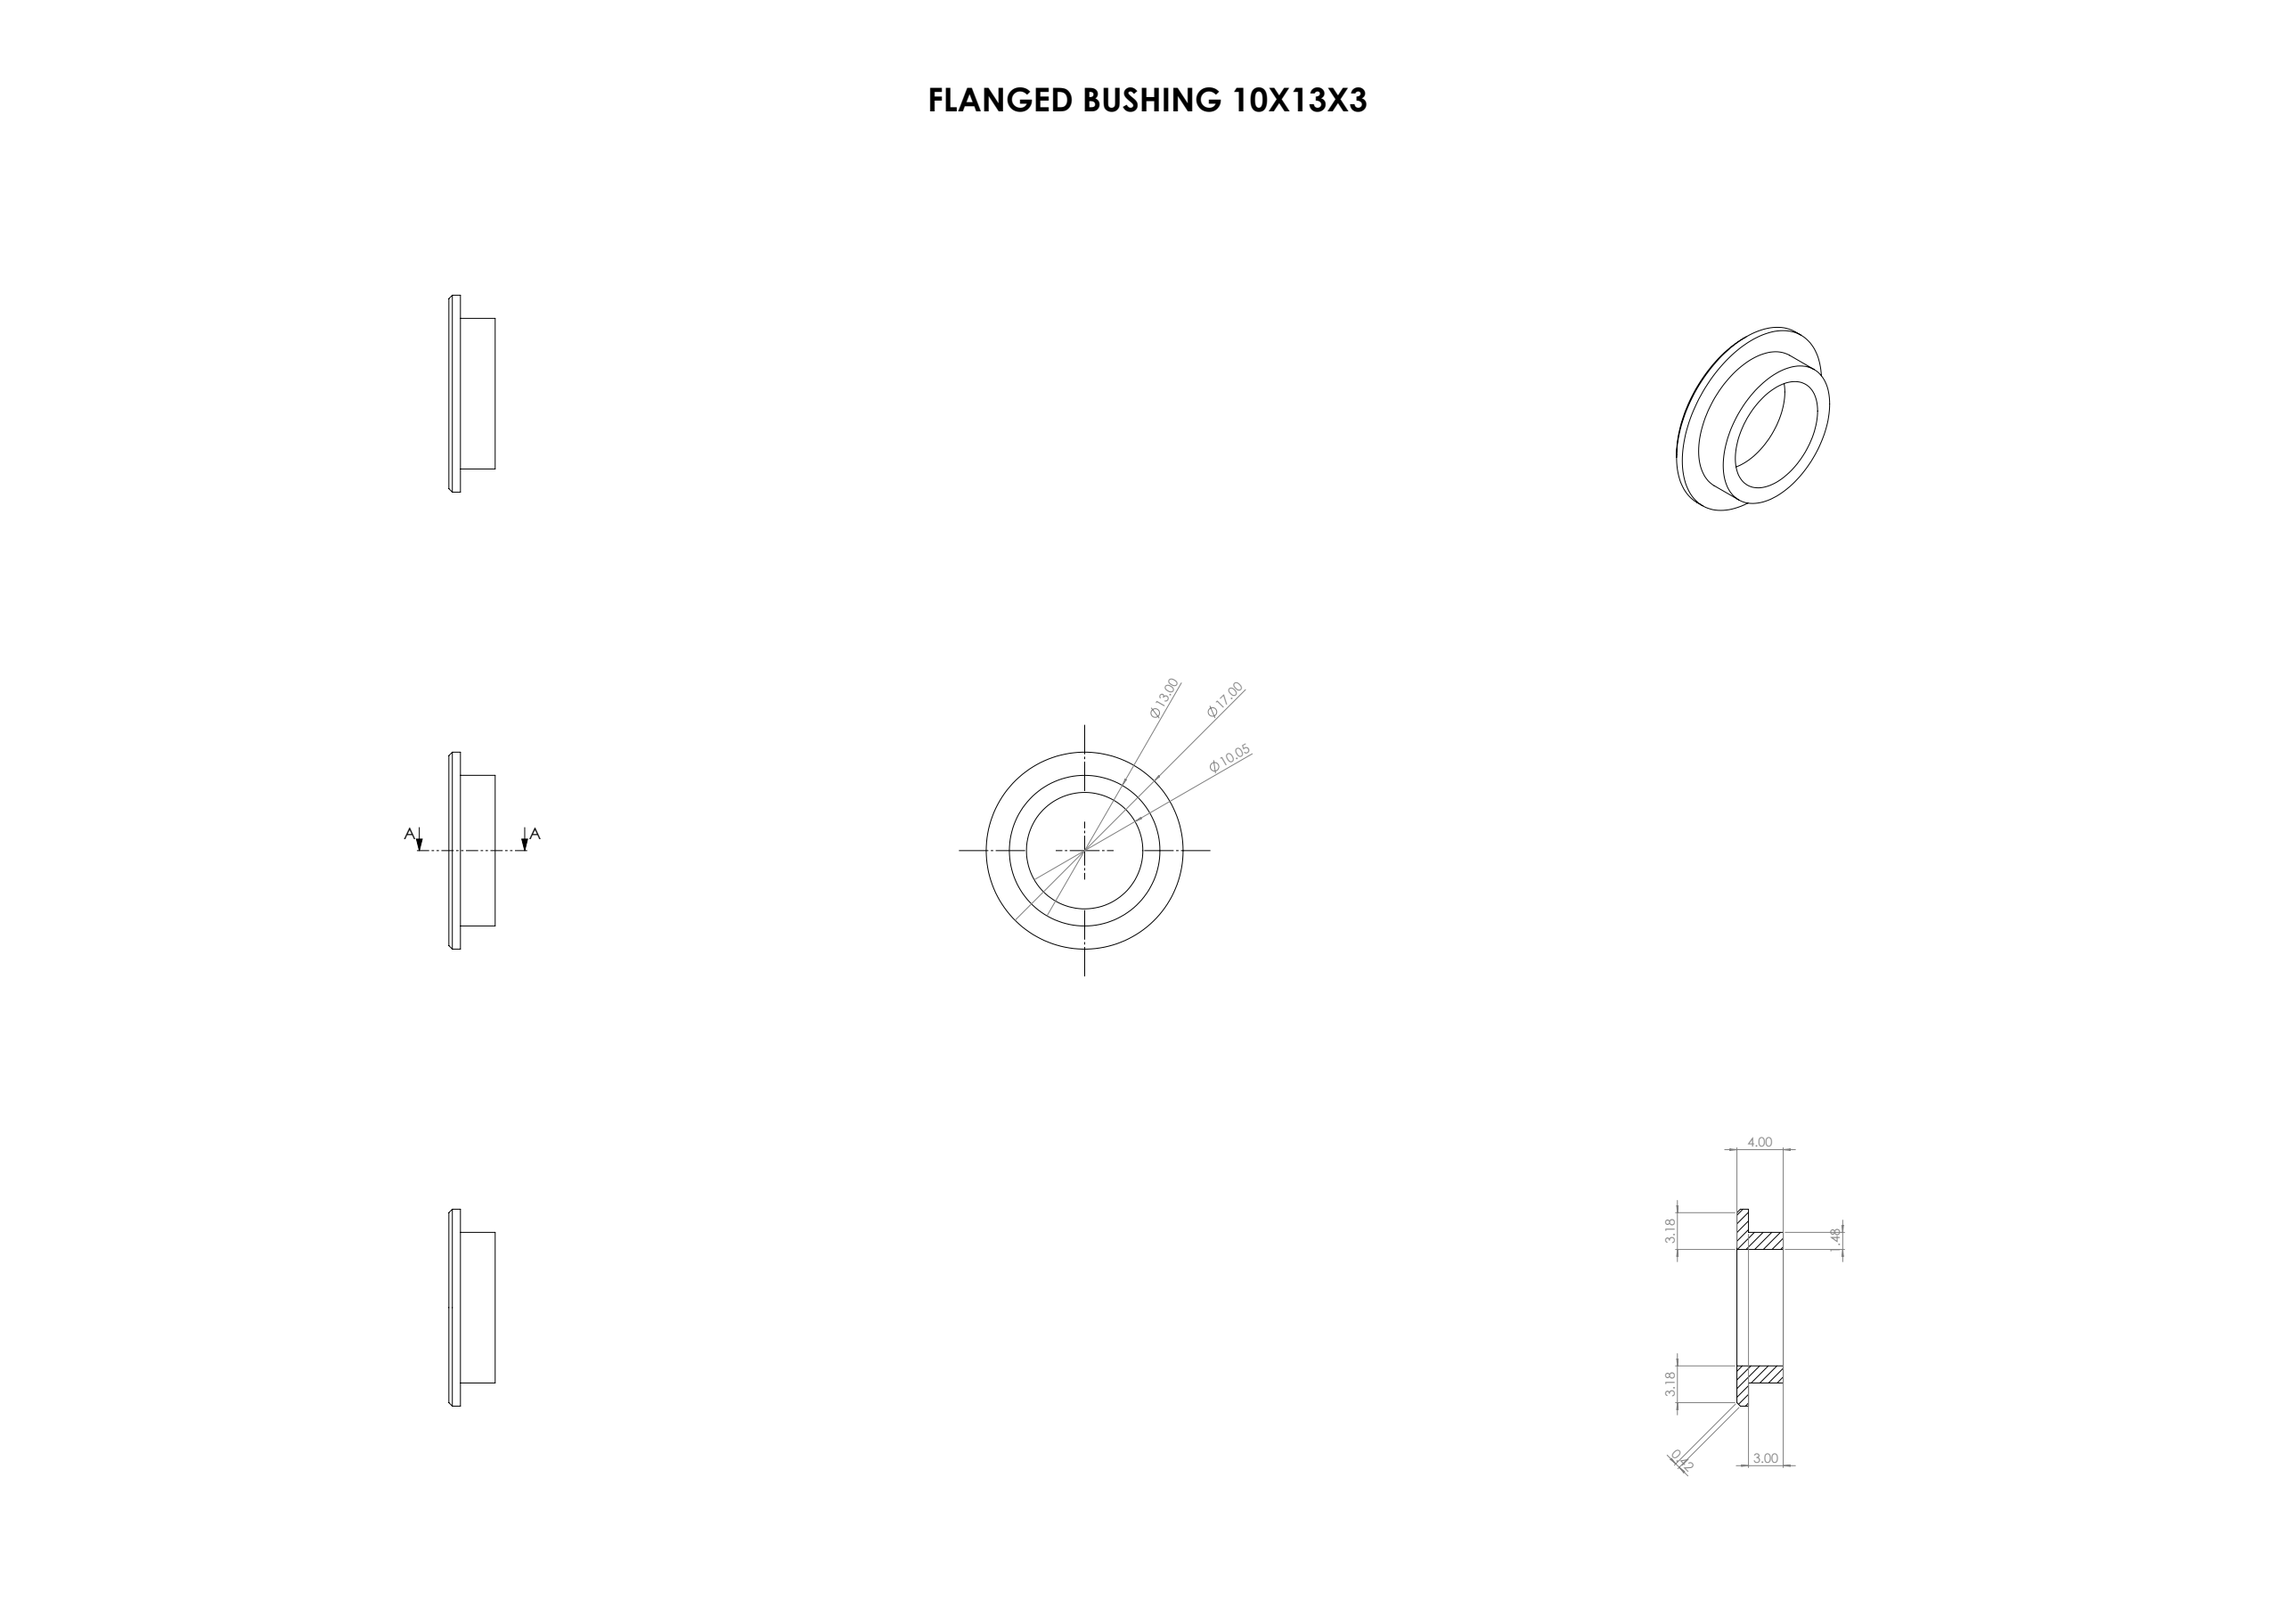
ISO-10303-21;
HEADER;
/* Generated by software containing ST-Developer
 * from STEP Tools, Inc. (www.steptools.com) 
 */

FILE_DESCRIPTION(
/* description */ (''),
/* implementation_level */ '2;1');

FILE_NAME(
/* name */ '08_Flanged_Bushing_10x13x3.step',
/* time_stamp */ '2026-10-21T01:59:45-07:00',
/* author */ (''),
/* organization */ (''),
/* preprocessor_version */ 'ST-DEVELOPER v20.2',
/* originating_system */ 'Autodesk Translation Framework v15.15.0.0',
/* authorisation */ '');

FILE_SCHEMA (('AUTOMOTIVE_DESIGN { 1 0 10303 214 3 1 1 }'));
ENDSEC;

DATA;
#10=MECHANICAL_DESIGN_GEOMETRIC_PRESENTATION_REPRESENTATION('',(#476),#18281);
#420=CONICAL_SURFACE('',#9714,8.35,0.785398163397449);
#445=SHAPE_REPRESENTATION_RELATIONSHIP('SRR','None',#18347,#458);
#458=ADVANCED_BREP_SHAPE_REPRESENTATION('',(#489),#18276);
#476=STYLED_ITEM('',(#18488),#489);
#489=MANIFOLD_SOLID_BREP('Body1',#9093);
#530=CYLINDRICAL_SURFACE('',#9720,8.5);
#531=CYLINDRICAL_SURFACE('',#9722,5.025);
#532=CYLINDRICAL_SURFACE('',#9726,6.5);
#620=FACE_BOUND('',#1771,.T.);
#621=FACE_BOUND('',#1775,.T.);
#622=FACE_BOUND('',#1778,.T.);
#755=CIRCLE('',#9715,8.5);
#756=CIRCLE('',#9716,8.5);
#757=CIRCLE('',#9717,8.2);
#758=CIRCLE('',#9719,5.025);
#759=CIRCLE('',#9721,8.5);
#760=CIRCLE('',#9723,5.025);
#761=CIRCLE('',#9725,6.5);
#762=CIRCLE('',#9727,6.5);
#1206=FACE_OUTER_BOUND('',#1769,.T.);
#1207=FACE_OUTER_BOUND('',#1770,.T.);
#1208=FACE_OUTER_BOUND('',#1772,.T.);
#1209=FACE_OUTER_BOUND('',#1773,.T.);
#1210=FACE_OUTER_BOUND('',#1774,.T.);
#1211=FACE_OUTER_BOUND('',#1776,.T.);
#1212=FACE_OUTER_BOUND('',#1777,.T.);
#1769=EDGE_LOOP('',(#7440,#7441,#7442,#7443,#7444));
#1770=EDGE_LOOP('',(#7445));
#1771=EDGE_LOOP('',(#7446));
#1772=EDGE_LOOP('',(#7447,#7448,#7449,#7450,#7451));
#1773=EDGE_LOOP('',(#7452,#7453,#7454,#7455));
#1774=EDGE_LOOP('',(#7456));
#1775=EDGE_LOOP('',(#7457));
#1776=EDGE_LOOP('',(#7458,#7459,#7460,#7461));
#1777=EDGE_LOOP('',(#7462));
#1778=EDGE_LOOP('',(#7463));
#2567=LINE('',#14541,#3412);
#2568=LINE('',#14549,#3413);
#2569=LINE('',#14553,#3414);
#2570=LINE('',#14560,#3415);
#3412=VECTOR('',#11551,8.35);
#3413=VECTOR('',#11562,8.5);
#3414=VECTOR('',#11567,5.025);
#3415=VECTOR('',#11576,6.5);
#4161=VERTEX_POINT('',#14536);
#4162=VERTEX_POINT('',#14537);
#4163=VERTEX_POINT('',#14540);
#4164=VERTEX_POINT('',#14544);
#4165=VERTEX_POINT('',#14547);
#4166=VERTEX_POINT('',#14551);
#4167=VERTEX_POINT('',#14555);
#4168=VERTEX_POINT('',#14558);
#5292=EDGE_CURVE('',#4161,#4162,#755,.T.);
#5293=EDGE_CURVE('',#4162,#4161,#756,.T.);
#5294=EDGE_CURVE('',#4161,#4163,#2567,.T.);
#5295=EDGE_CURVE('',#4163,#4163,#757,.T.);
#5296=EDGE_CURVE('',#4164,#4164,#758,.T.);
#5297=EDGE_CURVE('',#4165,#4165,#759,.T.);
#5298=EDGE_CURVE('',#4165,#4162,#2568,.T.);
#5299=EDGE_CURVE('',#4166,#4166,#760,.T.);
#5300=EDGE_CURVE('',#4166,#4164,#2569,.T.);
#5301=EDGE_CURVE('',#4167,#4167,#761,.T.);
#5302=EDGE_CURVE('',#4168,#4168,#762,.T.);
#5303=EDGE_CURVE('',#4168,#4167,#2570,.T.);
#7440=ORIENTED_EDGE('',*,*,#5292,.T.);
#7441=ORIENTED_EDGE('',*,*,#5293,.T.);
#7442=ORIENTED_EDGE('',*,*,#5294,.T.);
#7443=ORIENTED_EDGE('',*,*,#5295,.T.);
#7444=ORIENTED_EDGE('',*,*,#5294,.F.);
#7445=ORIENTED_EDGE('',*,*,#5295,.F.);
#7446=ORIENTED_EDGE('',*,*,#5296,.T.);
#7447=ORIENTED_EDGE('',*,*,#5297,.F.);
#7448=ORIENTED_EDGE('',*,*,#5298,.T.);
#7449=ORIENTED_EDGE('',*,*,#5292,.F.);
#7450=ORIENTED_EDGE('',*,*,#5293,.F.);
#7451=ORIENTED_EDGE('',*,*,#5298,.F.);
#7452=ORIENTED_EDGE('',*,*,#5299,.T.);
#7453=ORIENTED_EDGE('',*,*,#5300,.T.);
#7454=ORIENTED_EDGE('',*,*,#5296,.F.);
#7455=ORIENTED_EDGE('',*,*,#5300,.F.);
#7456=ORIENTED_EDGE('',*,*,#5297,.T.);
#7457=ORIENTED_EDGE('',*,*,#5301,.F.);
#7458=ORIENTED_EDGE('',*,*,#5302,.F.);
#7459=ORIENTED_EDGE('',*,*,#5303,.T.);
#7460=ORIENTED_EDGE('',*,*,#5301,.T.);
#7461=ORIENTED_EDGE('',*,*,#5303,.F.);
#7462=ORIENTED_EDGE('',*,*,#5302,.T.);
#7463=ORIENTED_EDGE('',*,*,#5299,.F.);
#8476=PLANE('',#9718);
#8477=PLANE('',#9724);
#8478=PLANE('',#9728);
#8927=ADVANCED_FACE('',(#1206),#420,.T.);
#8928=ADVANCED_FACE('',(#1207,#620),#8476,.T.);
#8929=ADVANCED_FACE('',(#1208),#530,.T.);
#8930=ADVANCED_FACE('',(#1209),#531,.F.);
#8931=ADVANCED_FACE('',(#1210,#621),#8477,.T.);
#8932=ADVANCED_FACE('',(#1211),#532,.T.);
#8933=ADVANCED_FACE('',(#1212,#622),#8478,.T.);
#9093=CLOSED_SHELL('',(#8927,#8928,#8929,#8930,#8931,#8932,#8933));
#9713=AXIS2_PLACEMENT_3D('',#14534,#11543,#11544);
#9714=AXIS2_PLACEMENT_3D('',#14535,#11545,#11546);
#9715=AXIS2_PLACEMENT_3D('',#14538,#11547,#11548);
#9716=AXIS2_PLACEMENT_3D('',#14539,#11549,#11550);
#9717=AXIS2_PLACEMENT_3D('',#14542,#11552,#11553);
#9718=AXIS2_PLACEMENT_3D('',#14543,#11554,#11555);
#9719=AXIS2_PLACEMENT_3D('',#14545,#11556,#11557);
#9720=AXIS2_PLACEMENT_3D('',#14546,#11558,#11559);
#9721=AXIS2_PLACEMENT_3D('',#14548,#11560,#11561);
#9722=AXIS2_PLACEMENT_3D('',#14550,#11563,#11564);
#9723=AXIS2_PLACEMENT_3D('',#14552,#11565,#11566);
#9724=AXIS2_PLACEMENT_3D('',#14554,#11568,#11569);
#9725=AXIS2_PLACEMENT_3D('',#14556,#11570,#11571);
#9726=AXIS2_PLACEMENT_3D('',#14557,#11572,#11573);
#9727=AXIS2_PLACEMENT_3D('',#14559,#11574,#11575);
#9728=AXIS2_PLACEMENT_3D('',#14561,#11577,#11578);
#11543=DIRECTION('axis',(0.,0.,1.));
#11544=DIRECTION('refdir',(1.,0.,0.));
#11545=DIRECTION('center_axis',(1.,0.,0.));
#11546=DIRECTION('ref_axis',(0.,-1.,0.));
#11547=DIRECTION('center_axis',(-1.,0.,0.));
#11548=DIRECTION('ref_axis',(0.,-1.,0.));
#11549=DIRECTION('center_axis',(-1.,0.,0.));
#11550=DIRECTION('ref_axis',(0.,-1.,0.));
#11551=DIRECTION('',(-0.707106781186547,-0.707106781186548,-8.65956056235494E-17));
#11552=DIRECTION('center_axis',(1.,0.,0.));
#11553=DIRECTION('ref_axis',(0.,-1.,0.));
#11554=DIRECTION('center_axis',(-1.,0.,0.));
#11555=DIRECTION('ref_axis',(0.,0.,1.));
#11556=DIRECTION('center_axis',(1.,0.,0.));
#11557=DIRECTION('ref_axis',(0.,0.,-1.));
#11558=DIRECTION('center_axis',(1.,0.,0.));
#11559=DIRECTION('ref_axis',(0.,1.,0.));
#11560=DIRECTION('center_axis',(1.,0.,0.));
#11561=DIRECTION('ref_axis',(0.,0.,-1.));
#11562=DIRECTION('',(-1.,0.,0.));
#11563=DIRECTION('center_axis',(1.,0.,0.));
#11564=DIRECTION('ref_axis',(0.,1.,0.));
#11565=DIRECTION('center_axis',(1.,0.,0.));
#11566=DIRECTION('ref_axis',(0.,0.,-1.));
#11567=DIRECTION('',(-1.,0.,0.));
#11568=DIRECTION('center_axis',(1.,0.,0.));
#11569=DIRECTION('ref_axis',(0.,0.,-1.));
#11570=DIRECTION('center_axis',(1.,0.,0.));
#11571=DIRECTION('ref_axis',(0.,0.,-1.));
#11572=DIRECTION('center_axis',(1.,0.,0.));
#11573=DIRECTION('ref_axis',(0.,1.,0.));
#11574=DIRECTION('center_axis',(1.,0.,0.));
#11575=DIRECTION('ref_axis',(0.,0.,-1.));
#11576=DIRECTION('',(-1.,0.,0.));
#11577=DIRECTION('center_axis',(1.,0.,0.));
#11578=DIRECTION('ref_axis',(0.,0.,-1.));
#14534=CARTESIAN_POINT('',(0.,0.,0.));
#14535=CARTESIAN_POINT('Origin',(-0.85,0.,0.));
#14536=CARTESIAN_POINT('',(-0.7,8.5,-1.04094977927525E-15));
#14537=CARTESIAN_POINT('',(-0.7,-8.5,-1.04094977927525E-15));
#14538=CARTESIAN_POINT('Origin',(-0.7,0.,0.));
#14539=CARTESIAN_POINT('Origin',(-0.7,0.,0.));
#14540=CARTESIAN_POINT('',(-1.,8.2,1.00421037530083E-15));
#14541=CARTESIAN_POINT('',(-0.85,8.35,1.02258007728804E-15));
#14542=CARTESIAN_POINT('Origin',(-1.,0.,0.));
#14543=CARTESIAN_POINT('Origin',(-1.,8.5,0.));
#14544=CARTESIAN_POINT('',(-1.,-5.025,-6.15385016571545E-16));
#14545=CARTESIAN_POINT('Origin',(-1.,0.,0.));
#14546=CARTESIAN_POINT('Origin',(-0.5,0.,0.));
#14547=CARTESIAN_POINT('',(0.,-8.5,-1.04094977927525E-15));
#14548=CARTESIAN_POINT('Origin',(0.,0.,0.));
#14549=CARTESIAN_POINT('',(-0.5,-8.5,-1.04094977927525E-15));
#14550=CARTESIAN_POINT('Origin',(1.,0.,0.));
#14551=CARTESIAN_POINT('',(3.,-5.025,-6.15385016571545E-16));
#14552=CARTESIAN_POINT('Origin',(3.,0.,0.));
#14553=CARTESIAN_POINT('',(1.,-5.025,-6.15385016571545E-16));
#14554=CARTESIAN_POINT('Origin',(0.,6.5,0.));
#14555=CARTESIAN_POINT('',(0.,-6.5,-7.9602041944578E-16));
#14556=CARTESIAN_POINT('Origin',(0.,0.,0.));
#14557=CARTESIAN_POINT('Origin',(1.5,0.,0.));
#14558=CARTESIAN_POINT('',(3.,-6.5,-7.9602041944578E-16));
#14559=CARTESIAN_POINT('Origin',(3.,0.,0.));
#14560=CARTESIAN_POINT('',(1.5,-6.5,-7.9602041944578E-16));
#14561=CARTESIAN_POINT('Origin',(3.,5.025,0.));
#18261=UNCERTAINTY_MEASURE_WITH_UNIT(LENGTH_MEASURE(0.01),#18282,
'DISTANCE_ACCURACY_VALUE',
'Maximum model space distance between geometric entities at asserted c
onnectivities');
#18266=UNCERTAINTY_MEASURE_WITH_UNIT(LENGTH_MEASURE(0.01),#18282,
'DISTANCE_ACCURACY_VALUE',
'Maximum model space distance between geometric entities at asserted c
onnectivities');
#18276=(
GEOMETRIC_REPRESENTATION_CONTEXT(3)
GLOBAL_UNCERTAINTY_ASSIGNED_CONTEXT((#18261))
GLOBAL_UNIT_ASSIGNED_CONTEXT((#18282,#18284,#18285))
REPRESENTATION_CONTEXT('','3D')
);
#18281=(
GEOMETRIC_REPRESENTATION_CONTEXT(3)
GLOBAL_UNCERTAINTY_ASSIGNED_CONTEXT((#18266))
GLOBAL_UNIT_ASSIGNED_CONTEXT((#18282,#18284,#18285))
REPRESENTATION_CONTEXT('','3D')
);
#18282=(
LENGTH_UNIT()
NAMED_UNIT(*)
SI_UNIT(.MILLI.,.METRE.)
);
#18284=(
NAMED_UNIT(*)
PLANE_ANGLE_UNIT()
SI_UNIT($,.RADIAN.)
);
#18285=(
NAMED_UNIT(*)
SI_UNIT($,.STERADIAN.)
SOLID_ANGLE_UNIT()
);
#18295=SHAPE_DEFINITION_REPRESENTATION(#18309,#18347);
#18309=PRODUCT_DEFINITION_SHAPE('',$,#18362);
#18347=SHAPE_REPRESENTATION('',(#9713),#18276);
#18352=PRODUCT_DEFINITION_CONTEXT('part definition',#18396,'design');
#18362=PRODUCT_DEFINITION('2026-10-20-13-03-22-090',
'08_Flanged_Bushing_10x13x3',#18376,#18352);
#18376=PRODUCT_DEFINITION_FORMATION('',$,#18407);
#18396=APPLICATION_CONTEXT(
'Core Data for Automotive Mechanical Design Process');
#18397=PRODUCT_CONTEXT('part definition',#18396,'mechanical');
#18407=PRODUCT('2026-10-20-13-03-22-090','08_Flanged_Bushing_10x13x3',$,
(#18397));
#18482=COLOUR_RGB('Off White',0.89,0.88,0.83);
#18483=FILL_AREA_STYLE_COLOUR('',#18482);
#18484=FILL_AREA_STYLE('',(#18483));
#18485=SURFACE_STYLE_FILL_AREA(#18484);
#18486=SURFACE_SIDE_STYLE('',(#18485));
#18487=SURFACE_STYLE_USAGE(.BOTH.,#18486);
#18488=PRESENTATION_STYLE_ASSIGNMENT((#18487));
ENDSEC;
END-ISO-10303-21;
